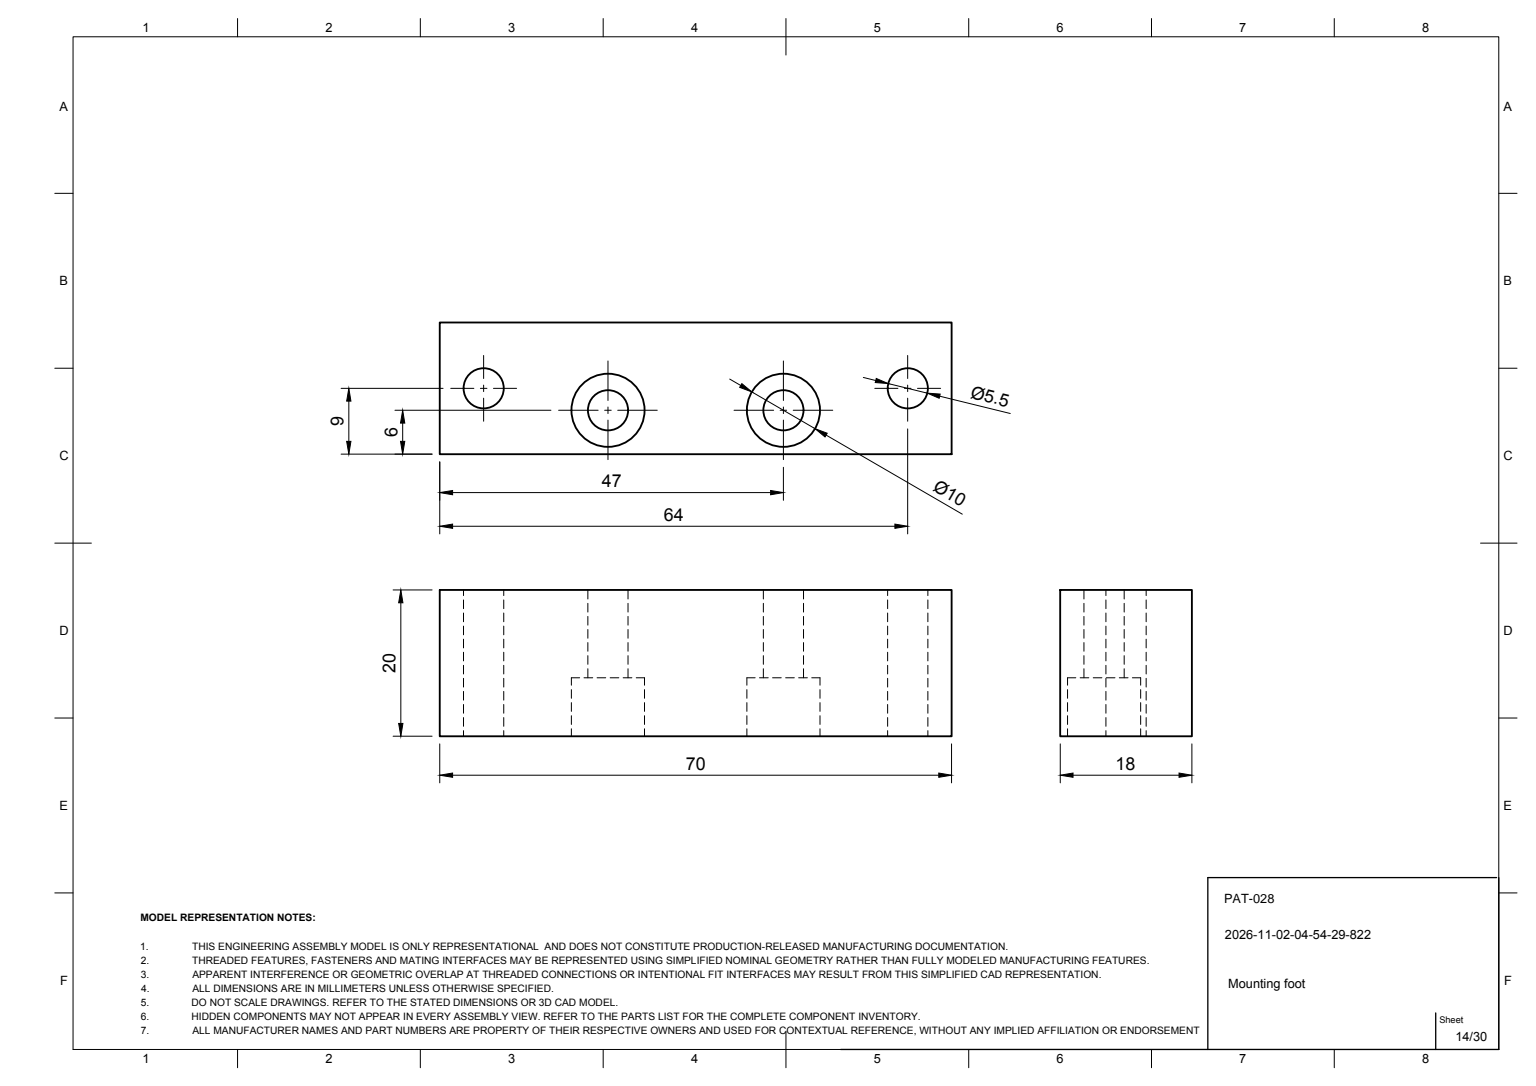
ISO-10303-21;
HEADER;
/* Generated by software containing ST-Developer
 * from STEP Tools, Inc. (www.steptools.com) 
 */

FILE_DESCRIPTION(
/* description */ ('Cylinder foot and clevis mount kit'),
/* implementation_level */ '2;1');

FILE_NAME(
/* name */ 'Mounting foot.step',
/* time_stamp */ '2026-10-27T20:10:43-07:00',
/* author */ (''),
/* organization */ (''),
/* preprocessor_version */ 'ST-DEVELOPER v20.2',
/* originating_system */ 'Autodesk Translation Framework v15.17.0.0',
/* authorisation */ '');

FILE_SCHEMA (('AUTOMOTIVE_DESIGN { 1 0 10303 214 3 1 1 }'));
ENDSEC;

DATA;
#10=MECHANICAL_DESIGN_GEOMETRIC_PRESENTATION_REPRESENTATION('',(#347),#9102);
#291=SHAPE_REPRESENTATION_RELATIONSHIP('SRR','None',#9238,#319);
#319=ADVANCED_BREP_SHAPE_REPRESENTATION('',(#375),#9081);
#347=STYLED_ITEM('',(#9453),#375);
#375=MANIFOLD_SOLID_BREP('Body1',#4933);
#446=FACE_BOUND('',#1204,.T.);
#447=FACE_BOUND('',#1207,.T.);
#448=FACE_BOUND('',#1215,.T.);
#449=FACE_BOUND('',#1216,.T.);
#450=FACE_BOUND('',#1217,.T.);
#451=FACE_BOUND('',#1218,.T.);
#452=FACE_BOUND('',#1220,.T.);
#453=FACE_BOUND('',#1221,.T.);
#454=FACE_BOUND('',#1222,.T.);
#455=FACE_BOUND('',#1223,.T.);
#597=PLANE('',#5551);
#598=PLANE('',#5556);
#599=PLANE('',#5562);
#600=PLANE('',#5563);
#601=PLANE('',#5564);
#602=PLANE('',#5565);
#603=PLANE('',#5566);
#604=PLANE('',#5567);
#840=FACE_OUTER_BOUND('',#1200,.T.);
#841=FACE_OUTER_BOUND('',#1201,.T.);
#842=FACE_OUTER_BOUND('',#1202,.T.);
#843=FACE_OUTER_BOUND('',#1203,.T.);
#844=FACE_OUTER_BOUND('',#1205,.T.);
#845=FACE_OUTER_BOUND('',#1206,.T.);
#846=FACE_OUTER_BOUND('',#1208,.T.);
#847=FACE_OUTER_BOUND('',#1209,.T.);
#848=FACE_OUTER_BOUND('',#1210,.T.);
#849=FACE_OUTER_BOUND('',#1211,.T.);
#850=FACE_OUTER_BOUND('',#1212,.T.);
#851=FACE_OUTER_BOUND('',#1213,.T.);
#852=FACE_OUTER_BOUND('',#1214,.T.);
#853=FACE_OUTER_BOUND('',#1219,.T.);
#1200=EDGE_LOOP('',(#3897,#3898,#3899,#3900));
#1201=EDGE_LOOP('',(#3901,#3902,#3903,#3904));
#1202=EDGE_LOOP('',(#3905,#3906,#3907,#3908));
#1203=EDGE_LOOP('',(#3909));
#1204=EDGE_LOOP('',(#3910));
#1205=EDGE_LOOP('',(#3911,#3912,#3913,#3914));
#1206=EDGE_LOOP('',(#3915));
#1207=EDGE_LOOP('',(#3916));
#1208=EDGE_LOOP('',(#3917,#3918,#3919,#3920));
#1209=EDGE_LOOP('',(#3921,#3922,#3923,#3924));
#1210=EDGE_LOOP('',(#3925,#3926,#3927,#3928));
#1211=EDGE_LOOP('',(#3929,#3930,#3931,#3932));
#1212=EDGE_LOOP('',(#3933,#3934,#3935,#3936));
#1213=EDGE_LOOP('',(#3937,#3938,#3939,#3940));
#1214=EDGE_LOOP('',(#3941,#3942,#3943,#3944));
#1215=EDGE_LOOP('',(#3945));
#1216=EDGE_LOOP('',(#3946));
#1217=EDGE_LOOP('',(#3947));
#1218=EDGE_LOOP('',(#3948));
#1219=EDGE_LOOP('',(#3949,#3950,#3951,#3952));
#1220=EDGE_LOOP('',(#3953));
#1221=EDGE_LOOP('',(#3954));
#1222=EDGE_LOOP('',(#3955));
#1223=EDGE_LOOP('',(#3956));
#1579=LINE('',#8130,#1928);
#1580=LINE('',#8136,#1929);
#1581=LINE('',#8142,#1930);
#1582=LINE('',#8151,#1931);
#1583=LINE('',#8158,#1932);
#1584=LINE('',#8162,#1933);
#1585=LINE('',#8167,#1934);
#1586=LINE('',#8169,#1935);
#1587=LINE('',#8171,#1936);
#1588=LINE('',#8172,#1937);
#1589=LINE('',#8175,#1938);
#1590=LINE('',#8177,#1939);
#1591=LINE('',#8178,#1940);
#1592=LINE('',#8181,#1941);
#1593=LINE('',#8183,#1942);
#1594=LINE('',#8184,#1943);
#1595=LINE('',#8186,#1944);
#1596=LINE('',#8187,#1945);
#1928=VECTOR('',#6622,0.275);
#1929=VECTOR('',#6629,0.275);
#1930=VECTOR('',#6636,0.5);
#1931=VECTOR('',#6647,0.5);
#1932=VECTOR('',#6656,0.275);
#1933=VECTOR('',#6661,0.275);
#1934=VECTOR('',#6666,1.);
#1935=VECTOR('',#6667,1.);
#1936=VECTOR('',#6668,1.);
#1937=VECTOR('',#6669,1.);
#1938=VECTOR('',#6672,1.);
#1939=VECTOR('',#6673,1.);
#1940=VECTOR('',#6674,1.);
#1941=VECTOR('',#6677,1.);
#1942=VECTOR('',#6678,1.);
#1943=VECTOR('',#6679,1.);
#1944=VECTOR('',#6682,1.);
#1945=VECTOR('',#6683,1.);
#2216=CIRCLE('',#5543,0.275);
#2217=CIRCLE('',#5544,0.275);
#2218=CIRCLE('',#5546,0.275);
#2219=CIRCLE('',#5547,0.275);
#2220=CIRCLE('',#5549,0.5);
#2221=CIRCLE('',#5550,0.5);
#2222=CIRCLE('',#5552,0.275);
#2223=CIRCLE('',#5554,0.5);
#2224=CIRCLE('',#5555,0.5);
#2225=CIRCLE('',#5557,0.275);
#2226=CIRCLE('',#5559,0.275);
#2227=CIRCLE('',#5561,0.275);
#2510=VERTEX_POINT('',#8127);
#2511=VERTEX_POINT('',#8129);
#2512=VERTEX_POINT('',#8133);
#2513=VERTEX_POINT('',#8135);
#2514=VERTEX_POINT('',#8139);
#2515=VERTEX_POINT('',#8141);
#2516=VERTEX_POINT('',#8145);
#2517=VERTEX_POINT('',#8148);
#2518=VERTEX_POINT('',#8150);
#2519=VERTEX_POINT('',#8154);
#2520=VERTEX_POINT('',#8157);
#2521=VERTEX_POINT('',#8161);
#2522=VERTEX_POINT('',#8165);
#2523=VERTEX_POINT('',#8166);
#2524=VERTEX_POINT('',#8168);
#2525=VERTEX_POINT('',#8170);
#2526=VERTEX_POINT('',#8174);
#2527=VERTEX_POINT('',#8176);
#2528=VERTEX_POINT('',#8180);
#2529=VERTEX_POINT('',#8182);
#3003=EDGE_CURVE('',#2510,#2510,#2216,.T.);
#3004=EDGE_CURVE('',#2510,#2511,#1579,.T.);
#3005=EDGE_CURVE('',#2511,#2511,#2217,.T.);
#3006=EDGE_CURVE('',#2512,#2512,#2218,.T.);
#3007=EDGE_CURVE('',#2512,#2513,#1580,.T.);
#3008=EDGE_CURVE('',#2513,#2513,#2219,.T.);
#3009=EDGE_CURVE('',#2514,#2514,#2220,.T.);
#3010=EDGE_CURVE('',#2514,#2515,#1581,.T.);
#3011=EDGE_CURVE('',#2515,#2515,#2221,.T.);
#3012=EDGE_CURVE('',#2516,#2516,#2222,.T.);
#3013=EDGE_CURVE('',#2517,#2517,#2223,.T.);
#3014=EDGE_CURVE('',#2517,#2518,#1582,.T.);
#3015=EDGE_CURVE('',#2518,#2518,#2224,.T.);
#3016=EDGE_CURVE('',#2519,#2519,#2225,.T.);
#3017=EDGE_CURVE('',#2516,#2520,#1583,.T.);
#3018=EDGE_CURVE('',#2520,#2520,#2226,.T.);
#3019=EDGE_CURVE('',#2519,#2521,#1584,.T.);
#3020=EDGE_CURVE('',#2521,#2521,#2227,.T.);
#3021=EDGE_CURVE('',#2522,#2523,#1585,.T.);
#3022=EDGE_CURVE('',#2523,#2524,#1586,.T.);
#3023=EDGE_CURVE('',#2525,#2524,#1587,.T.);
#3024=EDGE_CURVE('',#2522,#2525,#1588,.T.);
#3025=EDGE_CURVE('',#2526,#2522,#1589,.T.);
#3026=EDGE_CURVE('',#2527,#2525,#1590,.T.);
#3027=EDGE_CURVE('',#2526,#2527,#1591,.T.);
#3028=EDGE_CURVE('',#2528,#2526,#1592,.T.);
#3029=EDGE_CURVE('',#2529,#2527,#1593,.T.);
#3030=EDGE_CURVE('',#2528,#2529,#1594,.T.);
#3031=EDGE_CURVE('',#2523,#2528,#1595,.T.);
#3032=EDGE_CURVE('',#2524,#2529,#1596,.T.);
#3897=ORIENTED_EDGE('',*,*,#3003,.F.);
#3898=ORIENTED_EDGE('',*,*,#3004,.T.);
#3899=ORIENTED_EDGE('',*,*,#3005,.F.);
#3900=ORIENTED_EDGE('',*,*,#3004,.F.);
#3901=ORIENTED_EDGE('',*,*,#3006,.F.);
#3902=ORIENTED_EDGE('',*,*,#3007,.T.);
#3903=ORIENTED_EDGE('',*,*,#3008,.F.);
#3904=ORIENTED_EDGE('',*,*,#3007,.F.);
#3905=ORIENTED_EDGE('',*,*,#3009,.F.);
#3906=ORIENTED_EDGE('',*,*,#3010,.T.);
#3907=ORIENTED_EDGE('',*,*,#3011,.T.);
#3908=ORIENTED_EDGE('',*,*,#3010,.F.);
#3909=ORIENTED_EDGE('',*,*,#3011,.F.);
#3910=ORIENTED_EDGE('',*,*,#3012,.F.);
#3911=ORIENTED_EDGE('',*,*,#3013,.F.);
#3912=ORIENTED_EDGE('',*,*,#3014,.T.);
#3913=ORIENTED_EDGE('',*,*,#3015,.T.);
#3914=ORIENTED_EDGE('',*,*,#3014,.F.);
#3915=ORIENTED_EDGE('',*,*,#3015,.F.);
#3916=ORIENTED_EDGE('',*,*,#3016,.F.);
#3917=ORIENTED_EDGE('',*,*,#3012,.T.);
#3918=ORIENTED_EDGE('',*,*,#3017,.T.);
#3919=ORIENTED_EDGE('',*,*,#3018,.F.);
#3920=ORIENTED_EDGE('',*,*,#3017,.F.);
#3921=ORIENTED_EDGE('',*,*,#3016,.T.);
#3922=ORIENTED_EDGE('',*,*,#3019,.T.);
#3923=ORIENTED_EDGE('',*,*,#3020,.F.);
#3924=ORIENTED_EDGE('',*,*,#3019,.F.);
#3925=ORIENTED_EDGE('',*,*,#3021,.T.);
#3926=ORIENTED_EDGE('',*,*,#3022,.T.);
#3927=ORIENTED_EDGE('',*,*,#3023,.F.);
#3928=ORIENTED_EDGE('',*,*,#3024,.F.);
#3929=ORIENTED_EDGE('',*,*,#3025,.T.);
#3930=ORIENTED_EDGE('',*,*,#3024,.T.);
#3931=ORIENTED_EDGE('',*,*,#3026,.F.);
#3932=ORIENTED_EDGE('',*,*,#3027,.F.);
#3933=ORIENTED_EDGE('',*,*,#3028,.T.);
#3934=ORIENTED_EDGE('',*,*,#3027,.T.);
#3935=ORIENTED_EDGE('',*,*,#3029,.F.);
#3936=ORIENTED_EDGE('',*,*,#3030,.F.);
#3937=ORIENTED_EDGE('',*,*,#3031,.T.);
#3938=ORIENTED_EDGE('',*,*,#3030,.T.);
#3939=ORIENTED_EDGE('',*,*,#3032,.F.);
#3940=ORIENTED_EDGE('',*,*,#3022,.F.);
#3941=ORIENTED_EDGE('',*,*,#3032,.T.);
#3942=ORIENTED_EDGE('',*,*,#3029,.T.);
#3943=ORIENTED_EDGE('',*,*,#3026,.T.);
#3944=ORIENTED_EDGE('',*,*,#3023,.T.);
#3945=ORIENTED_EDGE('',*,*,#3005,.T.);
#3946=ORIENTED_EDGE('',*,*,#3008,.T.);
#3947=ORIENTED_EDGE('',*,*,#3018,.T.);
#3948=ORIENTED_EDGE('',*,*,#3020,.T.);
#3949=ORIENTED_EDGE('',*,*,#3031,.F.);
#3950=ORIENTED_EDGE('',*,*,#3021,.F.);
#3951=ORIENTED_EDGE('',*,*,#3025,.F.);
#3952=ORIENTED_EDGE('',*,*,#3028,.F.);
#3953=ORIENTED_EDGE('',*,*,#3003,.T.);
#3954=ORIENTED_EDGE('',*,*,#3006,.T.);
#3955=ORIENTED_EDGE('',*,*,#3009,.T.);
#3956=ORIENTED_EDGE('',*,*,#3013,.T.);
#4574=CYLINDRICAL_SURFACE('',#5542,0.275);
#4575=CYLINDRICAL_SURFACE('',#5545,0.275);
#4576=CYLINDRICAL_SURFACE('',#5548,0.5);
#4577=CYLINDRICAL_SURFACE('',#5553,0.5);
#4578=CYLINDRICAL_SURFACE('',#5558,0.275);
#4579=CYLINDRICAL_SURFACE('',#5560,0.275);
#4763=ADVANCED_FACE('',(#840),#4574,.F.);
#4764=ADVANCED_FACE('',(#841),#4575,.F.);
#4765=ADVANCED_FACE('',(#842),#4576,.F.);
#4766=ADVANCED_FACE('',(#843,#446),#597,.F.);
#4767=ADVANCED_FACE('',(#844),#4577,.F.);
#4768=ADVANCED_FACE('',(#845,#447),#598,.F.);
#4769=ADVANCED_FACE('',(#846),#4578,.F.);
#4770=ADVANCED_FACE('',(#847),#4579,.F.);
#4771=ADVANCED_FACE('',(#848),#599,.T.);
#4772=ADVANCED_FACE('',(#849),#600,.T.);
#4773=ADVANCED_FACE('',(#850),#601,.T.);
#4774=ADVANCED_FACE('',(#851),#602,.T.);
#4775=ADVANCED_FACE('',(#852,#448,#449,#450,#451),#603,.T.);
#4776=ADVANCED_FACE('',(#853,#452,#453,#454,#455),#604,.F.);
#4933=CLOSED_SHELL('',(#4763,#4764,#4765,#4766,#4767,#4768,#4769,#4770,
#4771,#4772,#4773,#4774,#4775,#4776));
#5541=AXIS2_PLACEMENT_3D('',#8125,#6616,#6617);
#5542=AXIS2_PLACEMENT_3D('',#8126,#6618,#6619);
#5543=AXIS2_PLACEMENT_3D('',#8128,#6620,#6621);
#5544=AXIS2_PLACEMENT_3D('',#8131,#6623,#6624);
#5545=AXIS2_PLACEMENT_3D('',#8132,#6625,#6626);
#5546=AXIS2_PLACEMENT_3D('',#8134,#6627,#6628);
#5547=AXIS2_PLACEMENT_3D('',#8137,#6630,#6631);
#5548=AXIS2_PLACEMENT_3D('',#8138,#6632,#6633);
#5549=AXIS2_PLACEMENT_3D('',#8140,#6634,#6635);
#5550=AXIS2_PLACEMENT_3D('',#8143,#6637,#6638);
#5551=AXIS2_PLACEMENT_3D('',#8144,#6639,#6640);
#5552=AXIS2_PLACEMENT_3D('',#8146,#6641,#6642);
#5553=AXIS2_PLACEMENT_3D('',#8147,#6643,#6644);
#5554=AXIS2_PLACEMENT_3D('',#8149,#6645,#6646);
#5555=AXIS2_PLACEMENT_3D('',#8152,#6648,#6649);
#5556=AXIS2_PLACEMENT_3D('',#8153,#6650,#6651);
#5557=AXIS2_PLACEMENT_3D('',#8155,#6652,#6653);
#5558=AXIS2_PLACEMENT_3D('',#8156,#6654,#6655);
#5559=AXIS2_PLACEMENT_3D('',#8159,#6657,#6658);
#5560=AXIS2_PLACEMENT_3D('',#8160,#6659,#6660);
#5561=AXIS2_PLACEMENT_3D('',#8163,#6662,#6663);
#5562=AXIS2_PLACEMENT_3D('',#8164,#6664,#6665);
#5563=AXIS2_PLACEMENT_3D('',#8173,#6670,#6671);
#5564=AXIS2_PLACEMENT_3D('',#8179,#6675,#6676);
#5565=AXIS2_PLACEMENT_3D('',#8185,#6680,#6681);
#5566=AXIS2_PLACEMENT_3D('',#8188,#6684,#6685);
#5567=AXIS2_PLACEMENT_3D('',#8189,#6686,#6687);
#6616=DIRECTION('axis',(0.,0.,1.));
#6617=DIRECTION('refdir',(1.,0.,0.));
#6618=DIRECTION('center_axis',(0.,0.,1.));
#6619=DIRECTION('ref_axis',(1.,0.,0.));
#6620=DIRECTION('center_axis',(0.,0.,1.));
#6621=DIRECTION('ref_axis',(1.,0.,0.));
#6622=DIRECTION('',(0.,0.,1.));
#6623=DIRECTION('center_axis',(0.,0.,-1.));
#6624=DIRECTION('ref_axis',(1.,0.,0.));
#6625=DIRECTION('center_axis',(0.,0.,1.));
#6626=DIRECTION('ref_axis',(1.,0.,0.));
#6627=DIRECTION('center_axis',(0.,0.,1.));
#6628=DIRECTION('ref_axis',(1.,0.,0.));
#6629=DIRECTION('',(0.,0.,1.));
#6630=DIRECTION('center_axis',(0.,0.,-1.));
#6631=DIRECTION('ref_axis',(1.,0.,0.));
#6632=DIRECTION('center_axis',(0.,0.,1.));
#6633=DIRECTION('ref_axis',(1.,0.,0.));
#6634=DIRECTION('center_axis',(0.,0.,1.));
#6635=DIRECTION('ref_axis',(1.,0.,0.));
#6636=DIRECTION('',(0.,0.,1.));
#6637=DIRECTION('center_axis',(0.,0.,1.));
#6638=DIRECTION('ref_axis',(1.,0.,0.));
#6639=DIRECTION('center_axis',(0.,0.,1.));
#6640=DIRECTION('ref_axis',(1.,0.,0.));
#6641=DIRECTION('center_axis',(0.,0.,-1.));
#6642=DIRECTION('ref_axis',(1.,0.,0.));
#6643=DIRECTION('center_axis',(0.,0.,1.));
#6644=DIRECTION('ref_axis',(1.,0.,0.));
#6645=DIRECTION('center_axis',(0.,0.,1.));
#6646=DIRECTION('ref_axis',(1.,0.,0.));
#6647=DIRECTION('',(0.,0.,1.));
#6648=DIRECTION('center_axis',(0.,0.,1.));
#6649=DIRECTION('ref_axis',(1.,0.,0.));
#6650=DIRECTION('center_axis',(0.,0.,1.));
#6651=DIRECTION('ref_axis',(1.,0.,0.));
#6652=DIRECTION('center_axis',(0.,0.,-1.));
#6653=DIRECTION('ref_axis',(1.,0.,0.));
#6654=DIRECTION('center_axis',(0.,0.,1.));
#6655=DIRECTION('ref_axis',(1.,0.,0.));
#6656=DIRECTION('',(0.,0.,1.));
#6657=DIRECTION('center_axis',(0.,0.,-1.));
#6658=DIRECTION('ref_axis',(1.,0.,0.));
#6659=DIRECTION('center_axis',(0.,0.,1.));
#6660=DIRECTION('ref_axis',(1.,0.,0.));
#6661=DIRECTION('',(0.,0.,1.));
#6662=DIRECTION('center_axis',(0.,0.,-1.));
#6663=DIRECTION('ref_axis',(1.,0.,0.));
#6664=DIRECTION('center_axis',(0.,1.,0.));
#6665=DIRECTION('ref_axis',(-1.,0.,0.));
#6666=DIRECTION('',(-1.,0.,0.));
#6667=DIRECTION('',(0.,0.,1.));
#6668=DIRECTION('',(-1.,0.,0.));
#6669=DIRECTION('',(0.,0.,1.));
#6670=DIRECTION('center_axis',(1.,0.,0.));
#6671=DIRECTION('ref_axis',(0.,1.,0.));
#6672=DIRECTION('',(0.,1.,0.));
#6673=DIRECTION('',(0.,1.,0.));
#6674=DIRECTION('',(0.,0.,1.));
#6675=DIRECTION('center_axis',(0.,-1.,0.));
#6676=DIRECTION('ref_axis',(1.,0.,0.));
#6677=DIRECTION('',(1.,0.,0.));
#6678=DIRECTION('',(1.,0.,0.));
#6679=DIRECTION('',(0.,0.,1.));
#6680=DIRECTION('center_axis',(-1.,0.,0.));
#6681=DIRECTION('ref_axis',(0.,-1.,0.));
#6682=DIRECTION('',(0.,-1.,0.));
#6683=DIRECTION('',(0.,-1.,0.));
#6684=DIRECTION('center_axis',(0.,0.,1.));
#6685=DIRECTION('ref_axis',(1.,0.,0.));
#6686=DIRECTION('center_axis',(0.,0.,1.));
#6687=DIRECTION('ref_axis',(1.,0.,0.));
#8125=CARTESIAN_POINT('',(0.,0.,0.));
#8126=CARTESIAN_POINT('Origin',(-2.9,0.9,-0.1));
#8127=CARTESIAN_POINT('',(-3.175,0.9,0.));
#8128=CARTESIAN_POINT('Origin',(-2.9,0.9,0.));
#8129=CARTESIAN_POINT('',(-3.175,0.9,2.));
#8130=CARTESIAN_POINT('',(-3.175,0.9,-0.1));
#8131=CARTESIAN_POINT('Origin',(-2.9,0.9,2.));
#8132=CARTESIAN_POINT('Origin',(2.9,0.9,-0.1));
#8133=CARTESIAN_POINT('',(2.625,0.9,0.));
#8134=CARTESIAN_POINT('Origin',(2.9,0.9,0.));
#8135=CARTESIAN_POINT('',(2.625,0.9,2.));
#8136=CARTESIAN_POINT('',(2.625,0.9,-0.1));
#8137=CARTESIAN_POINT('Origin',(2.9,0.9,2.));
#8138=CARTESIAN_POINT('Origin',(-1.2,0.6,-0.1));
#8139=CARTESIAN_POINT('',(-1.7,0.6,0.));
#8140=CARTESIAN_POINT('Origin',(-1.2,0.6,0.));
#8141=CARTESIAN_POINT('',(-1.7,0.6,0.8));
#8142=CARTESIAN_POINT('',(-1.7,0.6,-0.1));
#8143=CARTESIAN_POINT('Origin',(-1.2,0.6,0.8));
#8144=CARTESIAN_POINT('Origin',(-1.2,0.6,0.8));
#8145=CARTESIAN_POINT('',(-1.475,0.6,0.8));
#8146=CARTESIAN_POINT('Origin',(-1.2,0.6,0.8));
#8147=CARTESIAN_POINT('Origin',(1.2,0.6,-0.1));
#8148=CARTESIAN_POINT('',(0.7,0.6,0.));
#8149=CARTESIAN_POINT('Origin',(1.2,0.6,0.));
#8150=CARTESIAN_POINT('',(0.7,0.6,0.8));
#8151=CARTESIAN_POINT('',(0.7,0.6,-0.1));
#8152=CARTESIAN_POINT('Origin',(1.2,0.6,0.8));
#8153=CARTESIAN_POINT('Origin',(1.2,0.6,0.8));
#8154=CARTESIAN_POINT('',(0.925,0.6,0.8));
#8155=CARTESIAN_POINT('Origin',(1.2,0.6,0.8));
#8156=CARTESIAN_POINT('Origin',(-1.2,0.6,-0.1));
#8157=CARTESIAN_POINT('',(-1.475,0.6,2.));
#8158=CARTESIAN_POINT('',(-1.475,0.6,-0.1));
#8159=CARTESIAN_POINT('Origin',(-1.2,0.6,2.));
#8160=CARTESIAN_POINT('Origin',(1.2,0.6,-0.1));
#8161=CARTESIAN_POINT('',(0.925,0.6,2.));
#8162=CARTESIAN_POINT('',(0.925,0.6,-0.1));
#8163=CARTESIAN_POINT('Origin',(1.2,0.6,2.));
#8164=CARTESIAN_POINT('Origin',(3.5,1.8,0.));
#8165=CARTESIAN_POINT('',(3.5,1.8,0.));
#8166=CARTESIAN_POINT('',(-3.5,1.8,0.));
#8167=CARTESIAN_POINT('',(3.5,1.8,0.));
#8168=CARTESIAN_POINT('',(-3.5,1.8,2.));
#8169=CARTESIAN_POINT('',(-3.5,1.8,0.));
#8170=CARTESIAN_POINT('',(3.5,1.8,2.));
#8171=CARTESIAN_POINT('',(3.5,1.8,2.));
#8172=CARTESIAN_POINT('',(3.5,1.8,0.));
#8173=CARTESIAN_POINT('Origin',(3.5,0.,0.));
#8174=CARTESIAN_POINT('',(3.5,0.,0.));
#8175=CARTESIAN_POINT('',(3.5,0.,0.));
#8176=CARTESIAN_POINT('',(3.5,0.,2.));
#8177=CARTESIAN_POINT('',(3.5,0.,2.));
#8178=CARTESIAN_POINT('',(3.5,0.,0.));
#8179=CARTESIAN_POINT('Origin',(-3.5,0.,0.));
#8180=CARTESIAN_POINT('',(-3.5,0.,0.));
#8181=CARTESIAN_POINT('',(-3.5,0.,0.));
#8182=CARTESIAN_POINT('',(-3.5,0.,2.));
#8183=CARTESIAN_POINT('',(-3.5,0.,2.));
#8184=CARTESIAN_POINT('',(-3.5,0.,0.));
#8185=CARTESIAN_POINT('Origin',(-3.5,1.8,0.));
#8186=CARTESIAN_POINT('',(-3.5,1.8,0.));
#8187=CARTESIAN_POINT('',(-3.5,1.8,2.));
#8188=CARTESIAN_POINT('Origin',(0.,0.9,2.));
#8189=CARTESIAN_POINT('Origin',(0.,0.9,0.));
#9048=UNCERTAINTY_MEASURE_WITH_UNIT(LENGTH_MEASURE(0.001),#9103,
'DISTANCE_ACCURACY_VALUE',
'Maximum model space distance between geometric entities at asserted c
onnectivities');
#9069=UNCERTAINTY_MEASURE_WITH_UNIT(LENGTH_MEASURE(0.001),#9103,
'DISTANCE_ACCURACY_VALUE',
'Maximum model space distance between geometric entities at asserted c
onnectivities');
#9081=(
GEOMETRIC_REPRESENTATION_CONTEXT(3)
GLOBAL_UNCERTAINTY_ASSIGNED_CONTEXT((#9048))
GLOBAL_UNIT_ASSIGNED_CONTEXT((#9103,#9105,#9106))
REPRESENTATION_CONTEXT('','3D')
);
#9102=(
GEOMETRIC_REPRESENTATION_CONTEXT(3)
GLOBAL_UNCERTAINTY_ASSIGNED_CONTEXT((#9069))
GLOBAL_UNIT_ASSIGNED_CONTEXT((#9103,#9105,#9106))
REPRESENTATION_CONTEXT('','3D')
);
#9103=(
LENGTH_UNIT()
NAMED_UNIT(*)
SI_UNIT(.CENTI.,.METRE.)
);
#9105=(
NAMED_UNIT(*)
PLANE_ANGLE_UNIT()
SI_UNIT($,.RADIAN.)
);
#9106=(
NAMED_UNIT(*)
SI_UNIT($,.STERADIAN.)
SOLID_ANGLE_UNIT()
);
#9118=SHAPE_DEFINITION_REPRESENTATION(#9150,#9238);
#9150=PRODUCT_DEFINITION_SHAPE('',$,#9271);
#9238=SHAPE_REPRESENTATION('',(#5541),#9081);
#9259=PRODUCT_DEFINITION_CONTEXT('part definition',#9357,'design');
#9271=PRODUCT_DEFINITION('Mounting foot','Mounting foot',#9303,#9259);
#9303=PRODUCT_DEFINITION_FORMATION('',$,#9370);
#9357=APPLICATION_CONTEXT(
'Core Data for Automotive Mechanical Design Process');
#9358=PRODUCT_CONTEXT('part definition',#9357,'mechanical');
#9370=PRODUCT('Mounting foot','Mounting foot','Mounting foot',(#9358));
#9447=COLOUR_RGB('Sky Blue',0.24,0.69,0.87);
#9448=FILL_AREA_STYLE_COLOUR('',#9447);
#9449=FILL_AREA_STYLE('',(#9448));
#9450=SURFACE_STYLE_FILL_AREA(#9449);
#9451=SURFACE_SIDE_STYLE('',(#9450));
#9452=SURFACE_STYLE_USAGE(.BOTH.,#9451);
#9453=PRESENTATION_STYLE_ASSIGNMENT((#9452));
ENDSEC;
END-ISO-10303-21;
